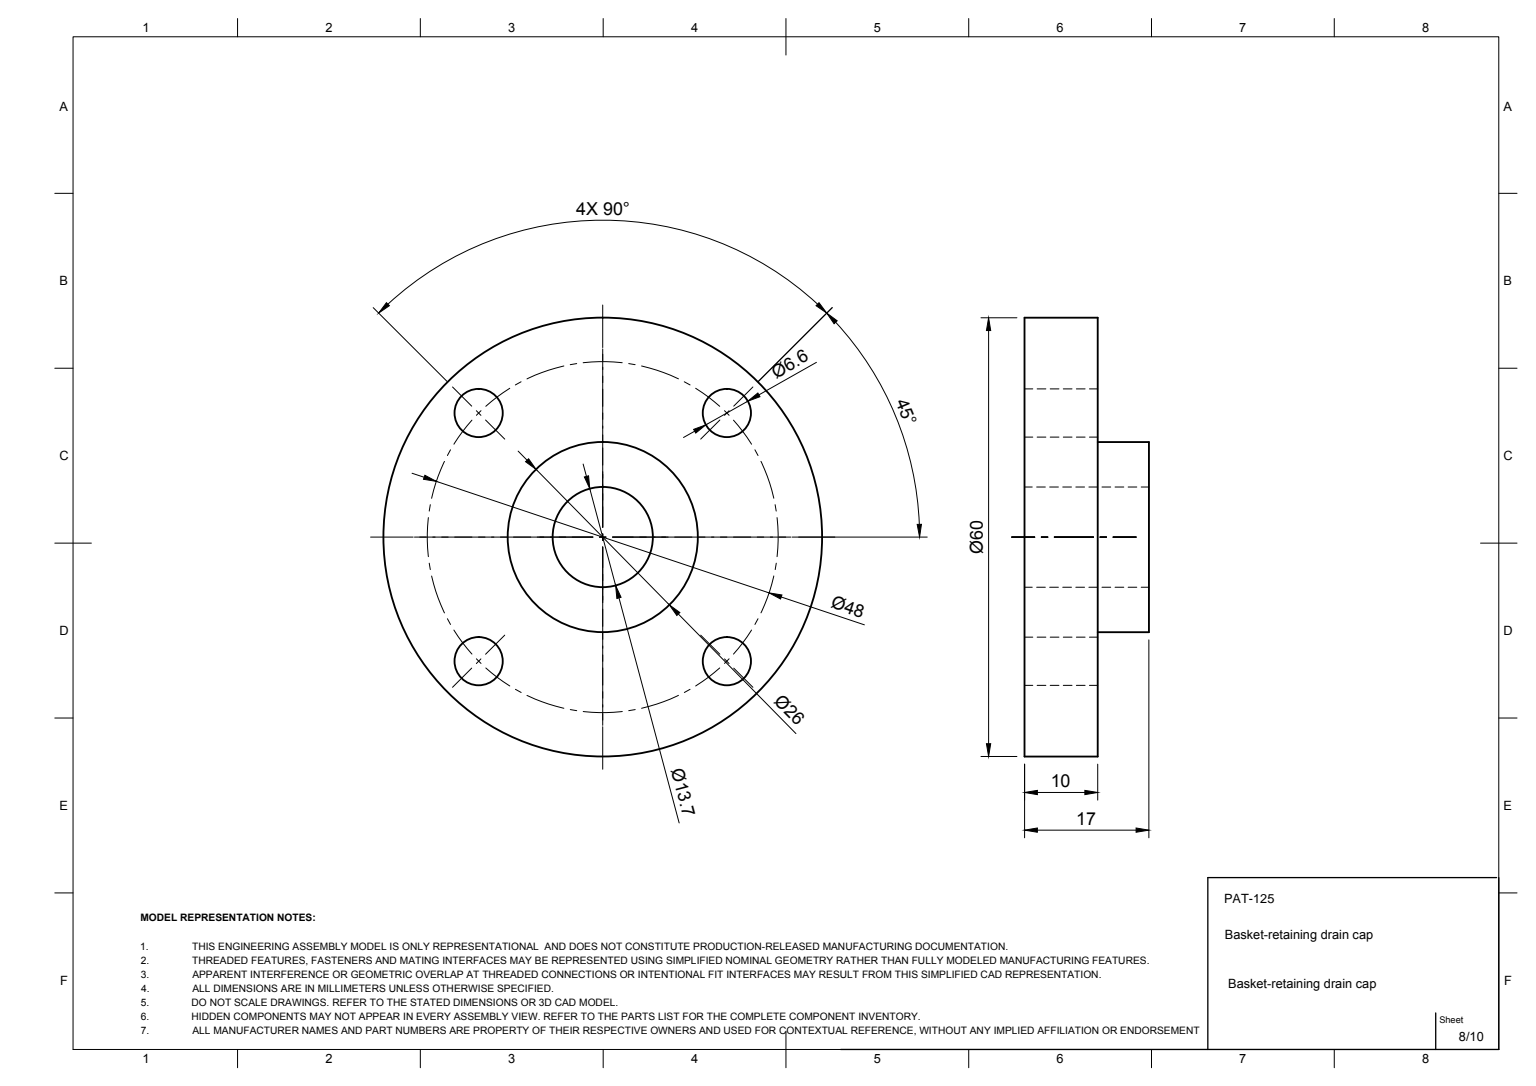
ISO-10303-21;
HEADER;
/* Generated by software containing ST-Developer
 * from STEP Tools, Inc. (www.steptools.com) 
 */

FILE_DESCRIPTION(
/* description */ ('Y-strainer with drain'),
/* implementation_level */ '2;1');

FILE_NAME(
/* name */ 'Basket-retaining drain cap.step',
/* time_stamp */ '2026-10-28T00:41:55-07:00',
/* author */ (''),
/* organization */ (''),
/* preprocessor_version */ 'ST-DEVELOPER v20.2',
/* originating_system */ 'Autodesk Translation Framework v15.17.0.0',
/* authorisation */ '');

FILE_SCHEMA (('AUTOMOTIVE_DESIGN { 1 0 10303 214 3 1 1 }'));
ENDSEC;

DATA;
#10=MECHANICAL_DESIGN_GEOMETRIC_PRESENTATION_REPRESENTATION('',(#98),#8864);
#80=SHAPE_REPRESENTATION_RELATIONSHIP('SRR','None',#8912,#89);
#89=ADVANCED_BREP_SHAPE_REPRESENTATION('',(#107),#8860);
#98=STYLED_ITEM('',(#9019),#107);
#107=MANIFOLD_SOLID_BREP('Body1',#3388);
#439=FACE_BOUND('',#899,.T.);
#440=FACE_BOUND('',#902,.T.);
#441=FACE_BOUND('',#903,.T.);
#442=FACE_BOUND('',#904,.T.);
#443=FACE_BOUND('',#905,.T.);
#444=FACE_BOUND('',#906,.T.);
#445=FACE_BOUND('',#908,.T.);
#446=FACE_BOUND('',#909,.T.);
#447=FACE_BOUND('',#910,.T.);
#448=FACE_BOUND('',#911,.T.);
#449=FACE_BOUND('',#912,.T.);
#487=PLANE('',#3688);
#488=PLANE('',#3692);
#489=PLANE('',#3693);
#620=FACE_OUTER_BOUND('',#892,.T.);
#621=FACE_OUTER_BOUND('',#893,.T.);
#622=FACE_OUTER_BOUND('',#894,.T.);
#623=FACE_OUTER_BOUND('',#895,.T.);
#624=FACE_OUTER_BOUND('',#896,.T.);
#625=FACE_OUTER_BOUND('',#897,.T.);
#626=FACE_OUTER_BOUND('',#898,.T.);
#627=FACE_OUTER_BOUND('',#900,.T.);
#628=FACE_OUTER_BOUND('',#901,.T.);
#629=FACE_OUTER_BOUND('',#907,.T.);
#892=EDGE_LOOP('',(#2930,#2931,#2932,#2933));
#893=EDGE_LOOP('',(#2934,#2935,#2936,#2937));
#894=EDGE_LOOP('',(#2938,#2939,#2940,#2941));
#895=EDGE_LOOP('',(#2942,#2943,#2944,#2945));
#896=EDGE_LOOP('',(#2946,#2947,#2948,#2949));
#897=EDGE_LOOP('',(#2950,#2951,#2952,#2953));
#898=EDGE_LOOP('',(#2954));
#899=EDGE_LOOP('',(#2955));
#900=EDGE_LOOP('',(#2956,#2957,#2958,#2959));
#901=EDGE_LOOP('',(#2960));
#902=EDGE_LOOP('',(#2961));
#903=EDGE_LOOP('',(#2962));
#904=EDGE_LOOP('',(#2963));
#905=EDGE_LOOP('',(#2964));
#906=EDGE_LOOP('',(#2965));
#907=EDGE_LOOP('',(#2966));
#908=EDGE_LOOP('',(#2967));
#909=EDGE_LOOP('',(#2968));
#910=EDGE_LOOP('',(#2969));
#911=EDGE_LOOP('',(#2970));
#912=EDGE_LOOP('',(#2971));
#1051=LINE('',#8603,#1214);
#1052=LINE('',#8609,#1215);
#1053=LINE('',#8615,#1216);
#1054=LINE('',#8621,#1217);
#1055=LINE('',#8627,#1218);
#1056=LINE('',#8633,#1219);
#1057=LINE('',#8640,#1220);
#1214=VECTOR('',#4219,0.33);
#1215=VECTOR('',#4226,0.33);
#1216=VECTOR('',#4233,0.33);
#1217=VECTOR('',#4240,0.33);
#1218=VECTOR('',#4247,0.685);
#1219=VECTOR('',#4254,1.3);
#1220=VECTOR('',#4263,3.);
#1347=CIRCLE('',#3671,0.33);
#1348=CIRCLE('',#3672,0.33);
#1349=CIRCLE('',#3674,0.33);
#1350=CIRCLE('',#3675,0.33);
#1351=CIRCLE('',#3677,0.33);
#1352=CIRCLE('',#3678,0.33);
#1353=CIRCLE('',#3680,0.33);
#1354=CIRCLE('',#3681,0.33);
#1355=CIRCLE('',#3683,0.685);
#1356=CIRCLE('',#3684,0.685);
#1357=CIRCLE('',#3686,1.3);
#1358=CIRCLE('',#3687,1.3);
#1359=CIRCLE('',#3690,3.);
#1360=CIRCLE('',#3691,3.);
#1653=VERTEX_POINT('',#8600);
#1654=VERTEX_POINT('',#8602);
#1655=VERTEX_POINT('',#8606);
#1656=VERTEX_POINT('',#8608);
#1657=VERTEX_POINT('',#8612);
#1658=VERTEX_POINT('',#8614);
#1659=VERTEX_POINT('',#8618);
#1660=VERTEX_POINT('',#8620);
#1661=VERTEX_POINT('',#8624);
#1662=VERTEX_POINT('',#8626);
#1663=VERTEX_POINT('',#8630);
#1664=VERTEX_POINT('',#8632);
#1665=VERTEX_POINT('',#8637);
#1666=VERTEX_POINT('',#8639);
#2089=EDGE_CURVE('',#1653,#1653,#1347,.T.);
#2090=EDGE_CURVE('',#1653,#1654,#1051,.T.);
#2091=EDGE_CURVE('',#1654,#1654,#1348,.T.);
#2092=EDGE_CURVE('',#1655,#1655,#1349,.T.);
#2093=EDGE_CURVE('',#1655,#1656,#1052,.T.);
#2094=EDGE_CURVE('',#1656,#1656,#1350,.T.);
#2095=EDGE_CURVE('',#1657,#1657,#1351,.T.);
#2096=EDGE_CURVE('',#1657,#1658,#1053,.T.);
#2097=EDGE_CURVE('',#1658,#1658,#1352,.T.);
#2098=EDGE_CURVE('',#1659,#1659,#1353,.T.);
#2099=EDGE_CURVE('',#1659,#1660,#1054,.T.);
#2100=EDGE_CURVE('',#1660,#1660,#1354,.T.);
#2101=EDGE_CURVE('',#1661,#1661,#1355,.T.);
#2102=EDGE_CURVE('',#1661,#1662,#1055,.T.);
#2103=EDGE_CURVE('',#1662,#1662,#1356,.T.);
#2104=EDGE_CURVE('',#1663,#1663,#1357,.T.);
#2105=EDGE_CURVE('',#1663,#1664,#1056,.T.);
#2106=EDGE_CURVE('',#1664,#1664,#1358,.T.);
#2107=EDGE_CURVE('',#1665,#1665,#1359,.T.);
#2108=EDGE_CURVE('',#1665,#1666,#1057,.T.);
#2109=EDGE_CURVE('',#1666,#1666,#1360,.T.);
#2930=ORIENTED_EDGE('',*,*,#2089,.F.);
#2931=ORIENTED_EDGE('',*,*,#2090,.T.);
#2932=ORIENTED_EDGE('',*,*,#2091,.F.);
#2933=ORIENTED_EDGE('',*,*,#2090,.F.);
#2934=ORIENTED_EDGE('',*,*,#2092,.F.);
#2935=ORIENTED_EDGE('',*,*,#2093,.T.);
#2936=ORIENTED_EDGE('',*,*,#2094,.F.);
#2937=ORIENTED_EDGE('',*,*,#2093,.F.);
#2938=ORIENTED_EDGE('',*,*,#2095,.F.);
#2939=ORIENTED_EDGE('',*,*,#2096,.T.);
#2940=ORIENTED_EDGE('',*,*,#2097,.F.);
#2941=ORIENTED_EDGE('',*,*,#2096,.F.);
#2942=ORIENTED_EDGE('',*,*,#2098,.F.);
#2943=ORIENTED_EDGE('',*,*,#2099,.T.);
#2944=ORIENTED_EDGE('',*,*,#2100,.F.);
#2945=ORIENTED_EDGE('',*,*,#2099,.F.);
#2946=ORIENTED_EDGE('',*,*,#2101,.F.);
#2947=ORIENTED_EDGE('',*,*,#2102,.T.);
#2948=ORIENTED_EDGE('',*,*,#2103,.F.);
#2949=ORIENTED_EDGE('',*,*,#2102,.F.);
#2950=ORIENTED_EDGE('',*,*,#2104,.F.);
#2951=ORIENTED_EDGE('',*,*,#2105,.T.);
#2952=ORIENTED_EDGE('',*,*,#2106,.T.);
#2953=ORIENTED_EDGE('',*,*,#2105,.F.);
#2954=ORIENTED_EDGE('',*,*,#2106,.F.);
#2955=ORIENTED_EDGE('',*,*,#2101,.T.);
#2956=ORIENTED_EDGE('',*,*,#2107,.F.);
#2957=ORIENTED_EDGE('',*,*,#2108,.T.);
#2958=ORIENTED_EDGE('',*,*,#2109,.T.);
#2959=ORIENTED_EDGE('',*,*,#2108,.F.);
#2960=ORIENTED_EDGE('',*,*,#2107,.T.);
#2961=ORIENTED_EDGE('',*,*,#2103,.T.);
#2962=ORIENTED_EDGE('',*,*,#2100,.T.);
#2963=ORIENTED_EDGE('',*,*,#2097,.T.);
#2964=ORIENTED_EDGE('',*,*,#2094,.T.);
#2965=ORIENTED_EDGE('',*,*,#2091,.T.);
#2966=ORIENTED_EDGE('',*,*,#2109,.F.);
#2967=ORIENTED_EDGE('',*,*,#2104,.T.);
#2968=ORIENTED_EDGE('',*,*,#2098,.T.);
#2969=ORIENTED_EDGE('',*,*,#2095,.T.);
#2970=ORIENTED_EDGE('',*,*,#2092,.T.);
#2971=ORIENTED_EDGE('',*,*,#2089,.T.);
#3218=CYLINDRICAL_SURFACE('',#3670,0.33);
#3219=CYLINDRICAL_SURFACE('',#3673,0.33);
#3220=CYLINDRICAL_SURFACE('',#3676,0.33);
#3221=CYLINDRICAL_SURFACE('',#3679,0.33);
#3222=CYLINDRICAL_SURFACE('',#3682,0.685);
#3223=CYLINDRICAL_SURFACE('',#3685,1.3);
#3224=CYLINDRICAL_SURFACE('',#3689,3.);
#3331=ADVANCED_FACE('',(#620),#3218,.F.);
#3332=ADVANCED_FACE('',(#621),#3219,.F.);
#3333=ADVANCED_FACE('',(#622),#3220,.F.);
#3334=ADVANCED_FACE('',(#623),#3221,.F.);
#3335=ADVANCED_FACE('',(#624),#3222,.F.);
#3336=ADVANCED_FACE('',(#625),#3223,.T.);
#3337=ADVANCED_FACE('',(#626,#439),#487,.F.);
#3338=ADVANCED_FACE('',(#627),#3224,.T.);
#3339=ADVANCED_FACE('',(#628,#440,#441,#442,#443,#444),#488,.T.);
#3340=ADVANCED_FACE('',(#629,#445,#446,#447,#448,#449),#489,.F.);
#3388=CLOSED_SHELL('',(#3331,#3332,#3333,#3334,#3335,#3336,#3337,#3338,
#3339,#3340));
#3669=AXIS2_PLACEMENT_3D('',#8598,#4213,#4214);
#3670=AXIS2_PLACEMENT_3D('',#8599,#4215,#4216);
#3671=AXIS2_PLACEMENT_3D('',#8601,#4217,#4218);
#3672=AXIS2_PLACEMENT_3D('',#8604,#4220,#4221);
#3673=AXIS2_PLACEMENT_3D('',#8605,#4222,#4223);
#3674=AXIS2_PLACEMENT_3D('',#8607,#4224,#4225);
#3675=AXIS2_PLACEMENT_3D('',#8610,#4227,#4228);
#3676=AXIS2_PLACEMENT_3D('',#8611,#4229,#4230);
#3677=AXIS2_PLACEMENT_3D('',#8613,#4231,#4232);
#3678=AXIS2_PLACEMENT_3D('',#8616,#4234,#4235);
#3679=AXIS2_PLACEMENT_3D('',#8617,#4236,#4237);
#3680=AXIS2_PLACEMENT_3D('',#8619,#4238,#4239);
#3681=AXIS2_PLACEMENT_3D('',#8622,#4241,#4242);
#3682=AXIS2_PLACEMENT_3D('',#8623,#4243,#4244);
#3683=AXIS2_PLACEMENT_3D('',#8625,#4245,#4246);
#3684=AXIS2_PLACEMENT_3D('',#8628,#4248,#4249);
#3685=AXIS2_PLACEMENT_3D('',#8629,#4250,#4251);
#3686=AXIS2_PLACEMENT_3D('',#8631,#4252,#4253);
#3687=AXIS2_PLACEMENT_3D('',#8634,#4255,#4256);
#3688=AXIS2_PLACEMENT_3D('',#8635,#4257,#4258);
#3689=AXIS2_PLACEMENT_3D('',#8636,#4259,#4260);
#3690=AXIS2_PLACEMENT_3D('',#8638,#4261,#4262);
#3691=AXIS2_PLACEMENT_3D('',#8641,#4264,#4265);
#3692=AXIS2_PLACEMENT_3D('',#8642,#4266,#4267);
#3693=AXIS2_PLACEMENT_3D('',#8643,#4268,#4269);
#4213=DIRECTION('axis',(0.,0.,1.));
#4214=DIRECTION('refdir',(1.,0.,0.));
#4215=DIRECTION('center_axis',(0.707106781186548,0.,-0.707106781186547));
#4216=DIRECTION('ref_axis',(-0.707106781186547,0.,-0.707106781186548));
#4217=DIRECTION('center_axis',(0.707106781186548,0.,-0.707106781186547));
#4218=DIRECTION('ref_axis',(-0.707106781186547,0.,-0.707106781186548));
#4219=DIRECTION('',(0.707106781186548,0.,-0.707106781186547));
#4220=DIRECTION('center_axis',(-0.707106781186548,0.,0.707106781186547));
#4221=DIRECTION('ref_axis',(-0.707106781186547,0.,-0.707106781186548));
#4222=DIRECTION('center_axis',(0.707106781186548,0.,-0.707106781186547));
#4223=DIRECTION('ref_axis',(-0.707106781186547,0.,-0.707106781186548));
#4224=DIRECTION('center_axis',(0.707106781186548,0.,-0.707106781186547));
#4225=DIRECTION('ref_axis',(-0.707106781186547,0.,-0.707106781186548));
#4226=DIRECTION('',(0.707106781186548,0.,-0.707106781186547));
#4227=DIRECTION('center_axis',(-0.707106781186548,0.,0.707106781186547));
#4228=DIRECTION('ref_axis',(-0.707106781186547,0.,-0.707106781186548));
#4229=DIRECTION('center_axis',(0.707106781186548,0.,-0.707106781186547));
#4230=DIRECTION('ref_axis',(-0.707106781186547,0.,-0.707106781186548));
#4231=DIRECTION('center_axis',(0.707106781186548,0.,-0.707106781186547));
#4232=DIRECTION('ref_axis',(-0.707106781186547,0.,-0.707106781186548));
#4233=DIRECTION('',(0.707106781186548,0.,-0.707106781186547));
#4234=DIRECTION('center_axis',(-0.707106781186548,0.,0.707106781186547));
#4235=DIRECTION('ref_axis',(-0.707106781186547,0.,-0.707106781186548));
#4236=DIRECTION('center_axis',(0.707106781186548,0.,-0.707106781186547));
#4237=DIRECTION('ref_axis',(-0.707106781186547,0.,-0.707106781186548));
#4238=DIRECTION('center_axis',(0.707106781186548,0.,-0.707106781186547));
#4239=DIRECTION('ref_axis',(-0.707106781186547,0.,-0.707106781186548));
#4240=DIRECTION('',(0.707106781186548,0.,-0.707106781186547));
#4241=DIRECTION('center_axis',(-0.707106781186548,0.,0.707106781186547));
#4242=DIRECTION('ref_axis',(-0.707106781186547,0.,-0.707106781186548));
#4243=DIRECTION('center_axis',(0.707106781186548,0.,-0.707106781186547));
#4244=DIRECTION('ref_axis',(-0.707106781186547,0.,-0.707106781186548));
#4245=DIRECTION('center_axis',(0.707106781186548,0.,-0.707106781186547));
#4246=DIRECTION('ref_axis',(-0.707106781186547,0.,-0.707106781186548));
#4247=DIRECTION('',(0.707106781186548,0.,-0.707106781186547));
#4248=DIRECTION('center_axis',(-0.707106781186548,0.,0.707106781186547));
#4249=DIRECTION('ref_axis',(-0.707106781186547,0.,-0.707106781186548));
#4250=DIRECTION('center_axis',(0.707106781186548,0.,-0.707106781186547));
#4251=DIRECTION('ref_axis',(-0.707106781186547,0.,-0.707106781186548));
#4252=DIRECTION('center_axis',(0.707106781186548,0.,-0.707106781186547));
#4253=DIRECTION('ref_axis',(-0.707106781186547,0.,-0.707106781186548));
#4254=DIRECTION('',(-0.707106781186548,0.,0.707106781186547));
#4255=DIRECTION('center_axis',(0.707106781186548,0.,-0.707106781186547));
#4256=DIRECTION('ref_axis',(-0.707106781186547,0.,-0.707106781186548));
#4257=DIRECTION('center_axis',(0.707106781186548,0.,-0.707106781186547));
#4258=DIRECTION('ref_axis',(-0.707106781186547,0.,-0.707106781186548));
#4259=DIRECTION('center_axis',(0.707106781186548,0.,-0.707106781186547));
#4260=DIRECTION('ref_axis',(-0.707106781186547,0.,-0.707106781186548));
#4261=DIRECTION('center_axis',(0.707106781186548,0.,-0.707106781186547));
#4262=DIRECTION('ref_axis',(-0.707106781186547,0.,-0.707106781186548));
#4263=DIRECTION('',(-0.707106781186548,0.,0.707106781186547));
#4264=DIRECTION('center_axis',(0.707106781186548,0.,-0.707106781186547));
#4265=DIRECTION('ref_axis',(-0.707106781186547,0.,-0.707106781186548));
#4266=DIRECTION('center_axis',(0.707106781186548,0.,-0.707106781186547));
#4267=DIRECTION('ref_axis',(-0.707106781186547,0.,-0.707106781186548));
#4268=DIRECTION('center_axis',(0.707106781186548,0.,-0.707106781186547));
#4269=DIRECTION('ref_axis',(-0.707106781186547,0.,-0.707106781186548));
#8598=CARTESIAN_POINT('',(0.,0.,0.));
#8599=CARTESIAN_POINT('Origin',(5.14974746830583,-1.69705627484771,3.25025253169417));
#8600=CARTESIAN_POINT('',(5.45380338421605,-1.69705627484771,3.41288709136707));
#8601=CARTESIAN_POINT('Origin',(5.22045814642449,-1.69705627484771,3.17954185357551));
#8602=CARTESIAN_POINT('',(6.1609101654026,-1.69705627484771,2.70578031018053));
#8603=CARTESIAN_POINT('',(5.38309270609739,-1.69705627484771,3.48359776948573));
#8604=CARTESIAN_POINT('Origin',(5.92756492761104,-1.69705627484771,2.47243507238896));
#8605=CARTESIAN_POINT('Origin',(5.14974746830583,1.69705627484771,3.25025253169417));
#8606=CARTESIAN_POINT('',(5.45380338421605,1.69705627484771,3.41288709136707));
#8607=CARTESIAN_POINT('Origin',(5.22045814642449,1.69705627484771,3.17954185357551));
#8608=CARTESIAN_POINT('',(6.1609101654026,1.69705627484771,2.70578031018053));
#8609=CARTESIAN_POINT('',(5.38309270609739,1.69705627484771,3.48359776948573));
#8610=CARTESIAN_POINT('Origin',(5.92756492761104,1.69705627484771,2.47243507238896));
#8611=CARTESIAN_POINT('Origin',(2.74974746830583,1.69705627484771,0.850252531694168));
#8612=CARTESIAN_POINT('',(3.05380338421605,1.69705627484771,1.01288709136707));
#8613=CARTESIAN_POINT('Origin',(2.82045814642449,1.69705627484771,0.779541853575513));
#8614=CARTESIAN_POINT('',(3.7609101654026,1.69705627484771,0.305780310180525));
#8615=CARTESIAN_POINT('',(2.98309270609739,1.69705627484771,1.08359776948573));
#8616=CARTESIAN_POINT('Origin',(3.52756492761104,1.69705627484771,0.0724350723889646));
#8617=CARTESIAN_POINT('Origin',(2.74974746830583,-1.69705627484771,0.850252531694168));
#8618=CARTESIAN_POINT('',(3.05380338421605,-1.69705627484771,1.01288709136707));
#8619=CARTESIAN_POINT('Origin',(2.82045814642449,-1.69705627484771,0.779541853575513));
#8620=CARTESIAN_POINT('',(3.7609101654026,-1.69705627484771,0.305780310180525));
#8621=CARTESIAN_POINT('',(2.98309270609739,-1.69705627484771,1.08359776948573));
#8622=CARTESIAN_POINT('Origin',(3.52756492761104,-1.69705627484771,0.0724350723889646));
#8623=CARTESIAN_POINT('Origin',(3.45477272147525,0.,2.54522727852475));
#8624=CARTESIAN_POINT('',(4.00985154470669,-8.38883057415937E-17,2.95888474551888));
#8625=CARTESIAN_POINT('Origin',(3.5254833995939,0.,2.4745166004061));
#8626=CARTESIAN_POINT('',(5.21193307272382,8.38883057415937E-17,1.75680321750175));
#8627=CARTESIAN_POINT('',(3.93914086658804,-8.38883057415937E-17,3.02959542363754));
#8628=CARTESIAN_POINT('Origin',(4.72756492761104,0.,1.27243507238896));
#8629=CARTESIAN_POINT('Origin',(3.5254833995939,0.,2.4745166004061));
#8630=CARTESIAN_POINT('',(4.939696961967,-1.59204083889156E-16,2.89878066911802));
#8631=CARTESIAN_POINT('Origin',(4.02045814642449,0.,1.97954185357551));
#8632=CARTESIAN_POINT('',(4.44472221513642,-1.59204083889156E-16,3.39375541594861));
#8633=CARTESIAN_POINT('',(4.44472221513642,-1.59204083889156E-16,3.39375541594861));
#8634=CARTESIAN_POINT('Origin',(3.5254833995939,0.,2.4745166004061));
#8635=CARTESIAN_POINT('Origin',(3.5254833995939,0.,2.4745166004061));
#8636=CARTESIAN_POINT('Origin',(4.02045814642449,0.,1.97954185357551));
#8637=CARTESIAN_POINT('',(6.84888527117068,-3.67394039744206E-16,3.39375541594861));
#8638=CARTESIAN_POINT('Origin',(4.72756492761104,0.,1.27243507238896));
#8639=CARTESIAN_POINT('',(6.14177848998413,-3.67394039744206E-16,4.10086219713516));
#8640=CARTESIAN_POINT('',(6.14177848998413,-3.67394039744206E-16,4.10086219713516));
#8641=CARTESIAN_POINT('Origin',(4.02045814642449,0.,1.97954185357551));
#8642=CARTESIAN_POINT('Origin',(4.72756492761104,0.,1.27243507238896));
#8643=CARTESIAN_POINT('Origin',(4.02045814642449,0.,1.97954185357551));
#8848=UNCERTAINTY_MEASURE_WITH_UNIT(LENGTH_MEASURE(0.001),#8865,
'DISTANCE_ACCURACY_VALUE',
'Maximum model space distance between geometric entities at asserted c
onnectivities');
#8852=UNCERTAINTY_MEASURE_WITH_UNIT(LENGTH_MEASURE(0.001),#8865,
'DISTANCE_ACCURACY_VALUE',
'Maximum model space distance between geometric entities at asserted c
onnectivities');
#8860=(
GEOMETRIC_REPRESENTATION_CONTEXT(3)
GLOBAL_UNCERTAINTY_ASSIGNED_CONTEXT((#8848))
GLOBAL_UNIT_ASSIGNED_CONTEXT((#8865,#8867,#8868))
REPRESENTATION_CONTEXT('','3D')
);
#8864=(
GEOMETRIC_REPRESENTATION_CONTEXT(3)
GLOBAL_UNCERTAINTY_ASSIGNED_CONTEXT((#8852))
GLOBAL_UNIT_ASSIGNED_CONTEXT((#8865,#8867,#8868))
REPRESENTATION_CONTEXT('','3D')
);
#8865=(
LENGTH_UNIT()
NAMED_UNIT(*)
SI_UNIT(.CENTI.,.METRE.)
);
#8867=(
NAMED_UNIT(*)
PLANE_ANGLE_UNIT()
SI_UNIT($,.RADIAN.)
);
#8868=(
NAMED_UNIT(*)
SI_UNIT($,.STERADIAN.)
SOLID_ANGLE_UNIT()
);
#8876=SHAPE_DEFINITION_REPRESENTATION(#8887,#8912);
#8887=PRODUCT_DEFINITION_SHAPE('',$,#8924);
#8912=SHAPE_REPRESENTATION('',(#3669),#8860);
#8916=PRODUCT_DEFINITION_CONTEXT('part definition',#8951,'design');
#8924=PRODUCT_DEFINITION('Basket-retaining drain cap',
'Basket-retaining drain cap',#8935,#8916);
#8935=PRODUCT_DEFINITION_FORMATION('',$,#8960);
#8951=APPLICATION_CONTEXT(
'Core Data for Automotive Mechanical Design Process');
#8952=PRODUCT_CONTEXT('part definition',#8951,'mechanical');
#8960=PRODUCT('Basket-retaining drain cap','Basket-retaining drain cap',
'Basket-retaining drain cap',(#8952));
#9013=COLOUR_RGB('Light Blue',0.38,0.62,0.78);
#9014=FILL_AREA_STYLE_COLOUR('',#9013);
#9015=FILL_AREA_STYLE('',(#9014));
#9016=SURFACE_STYLE_FILL_AREA(#9015);
#9017=SURFACE_SIDE_STYLE('',(#9016));
#9018=SURFACE_STYLE_USAGE(.BOTH.,#9017);
#9019=PRESENTATION_STYLE_ASSIGNMENT((#9018));
ENDSEC;
END-ISO-10303-21;
